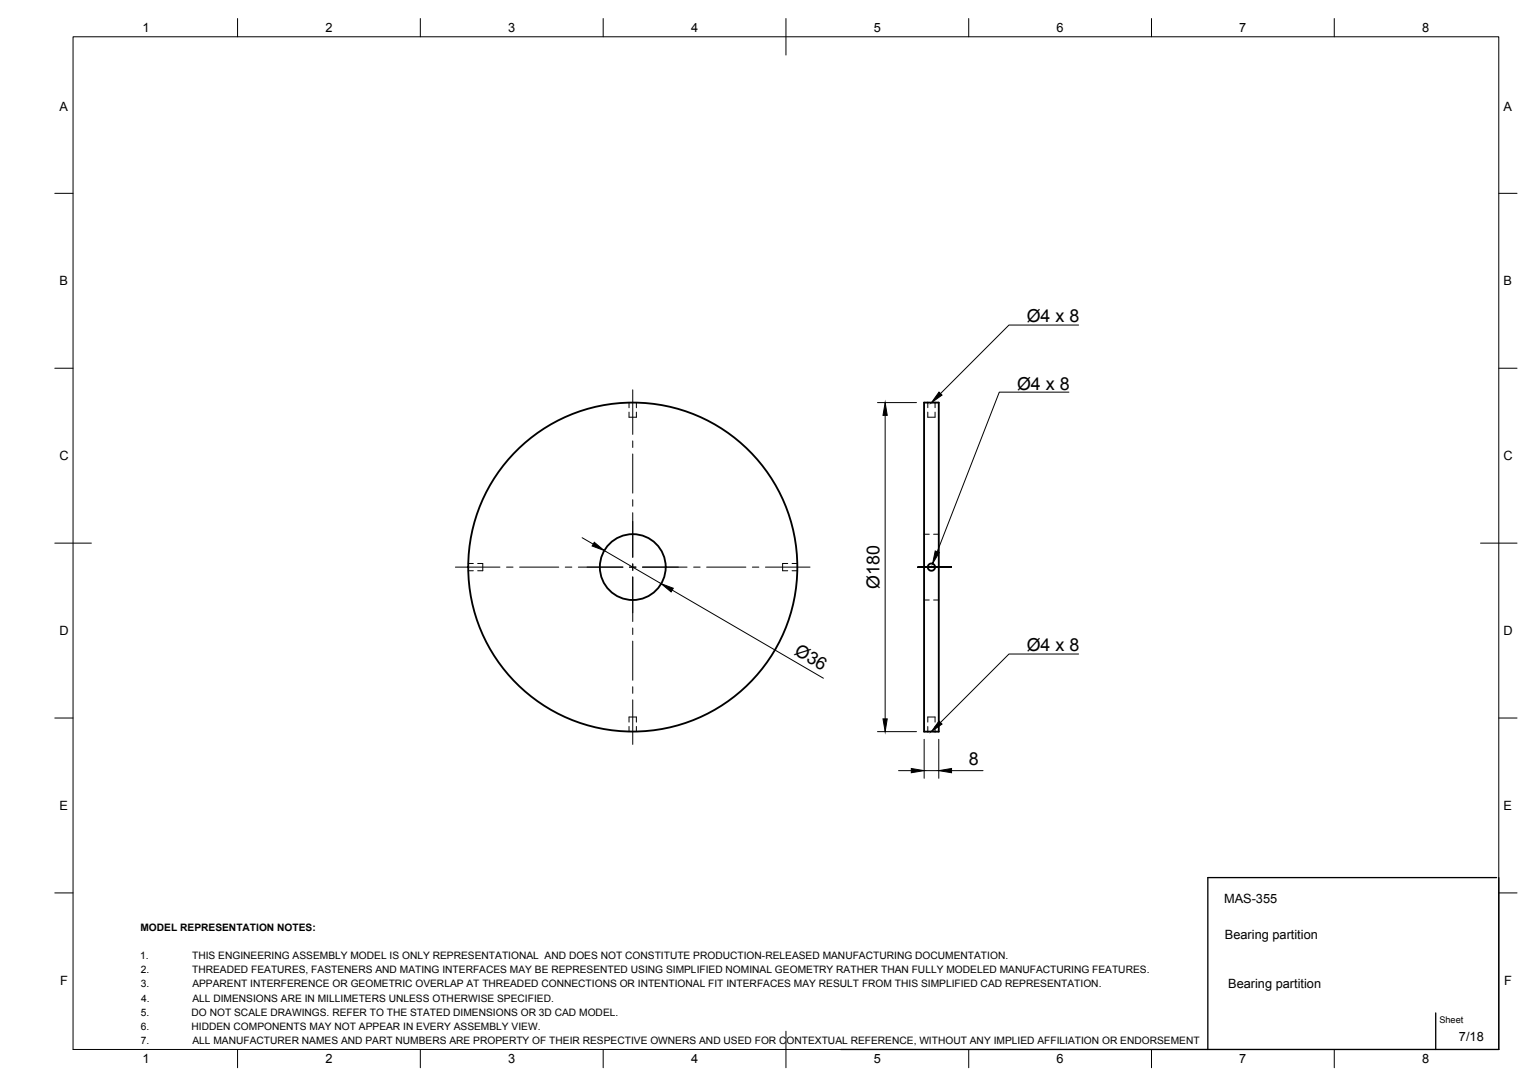
ISO-10303-21;
HEADER;
/* Generated by software containing ST-Developer
 * from STEP Tools, Inc. (www.steptools.com) 
 */

FILE_DESCRIPTION(
/* description */ ('Independent two-stage fixed-ring planetary gearbox,24/24/72 teeth,mod
ule2,20deg involutes,three planets per stage,4:1 x4:1=16:1. Native cut
-space/fillet/pattern tooth profiles derived from reusable gear blanks
; shared sun/planet/ring/carrier parts across both stages. Captured br
onze-journal input/carriers, headed retained planet pins, keyed inters
tage drive and modular keyed output interface. Native ideal gear links
; no torque, precision grade, production backlash/fits, lubrication, s
peed or life rating.'),
/* implementation_level */ '2;1');

FILE_NAME(
/* name */ 'Bearing partition.step',
/* time_stamp */ '2026-11-08T19:10:00-08:00',
/* author */ (''),
/* organization */ (''),
/* preprocessor_version */ 'ST-DEVELOPER v20.2',
/* originating_system */ 'Autodesk Translation Framework v15.17.0.0',
/* authorisation */ '');

FILE_SCHEMA (('AUTOMOTIVE_DESIGN { 1 0 10303 214 3 1 1 }'));
ENDSEC;

DATA;
#10=MECHANICAL_DESIGN_GEOMETRIC_PRESENTATION_REPRESENTATION('',(#1164),#259224);
#1124=SHAPE_REPRESENTATION_RELATIONSHIP('SRR','None',#259371,#1144);
#1144=ADVANCED_BREP_SHAPE_REPRESENTATION('',(#1184),#259205);
#1164=STYLED_ITEM('',(#259480),#1184);
#1184=MANIFOLD_SOLID_BREP('Body1',#25151);
#1242=FACE_BOUND('',#3407,.T.);
#1243=FACE_BOUND('',#3408,.T.);
#1244=FACE_BOUND('',#3409,.T.);
#1245=FACE_BOUND('',#3411,.T.);
#1246=FACE_BOUND('',#3413,.T.);
#1501=PLANE('',#25760);
#1502=PLANE('',#25763);
#1503=PLANE('',#25766);
#1504=PLANE('',#25769);
#1505=PLANE('',#25776);
#1506=PLANE('',#25777);
#2012=FACE_OUTER_BOUND('',#3397,.T.);
#2013=FACE_OUTER_BOUND('',#3398,.T.);
#2014=FACE_OUTER_BOUND('',#3399,.T.);
#2015=FACE_OUTER_BOUND('',#3400,.T.);
#2016=FACE_OUTER_BOUND('',#3401,.T.);
#2017=FACE_OUTER_BOUND('',#3402,.T.);
#2018=FACE_OUTER_BOUND('',#3403,.T.);
#2019=FACE_OUTER_BOUND('',#3404,.T.);
#2020=FACE_OUTER_BOUND('',#3405,.T.);
#2021=FACE_OUTER_BOUND('',#3406,.T.);
#2022=FACE_OUTER_BOUND('',#3410,.T.);
#2023=FACE_OUTER_BOUND('',#3412,.T.);
#3397=EDGE_LOOP('',(#17302,#17303,#17304,#17305,#17306));
#3398=EDGE_LOOP('',(#17307));
#3399=EDGE_LOOP('',(#17308,#17309,#17310,#17311,#17312));
#3400=EDGE_LOOP('',(#17313));
#3401=EDGE_LOOP('',(#17314,#17315,#17316,#17317,#17318,#17319));
#3402=EDGE_LOOP('',(#17320));
#3403=EDGE_LOOP('',(#17321,#17322,#17323,#17324,#17325,#17326));
#3404=EDGE_LOOP('',(#17327));
#3405=EDGE_LOOP('',(#17328,#17329,#17330,#17331));
#3406=EDGE_LOOP('',(#17332,#17333,#17334,#17335,#17336,#17337,#17338,#17339,
#17340));
#3407=EDGE_LOOP('',(#17341,#17342));
#3408=EDGE_LOOP('',(#17343,#17344));
#3409=EDGE_LOOP('',(#17345,#17346,#17347));
#3410=EDGE_LOOP('',(#17348));
#3411=EDGE_LOOP('',(#17349));
#3412=EDGE_LOOP('',(#17350));
#3413=EDGE_LOOP('',(#17351));
#4571=CIRCLE('',#25759,2.);
#4572=CIRCLE('',#25762,2.);
#4573=CIRCLE('',#25765,2.);
#4574=CIRCLE('',#25768,2.);
#4575=CIRCLE('',#25771,18.);
#4576=CIRCLE('',#25772,18.);
#4577=CIRCLE('',#25774,90.);
#4578=CIRCLE('',#25775,90.);
#5983=B_SPLINE_CURVE_WITH_KNOTS('',3,(#52036,#52037,#52038,#52039,#52040,
#52041,#52042,#52043,#52044,#52045,#52046,#52047,#52048,#52049,#52050,#52051,
#52052,#52053),.UNSPECIFIED.,.F.,.F.,(4,2,2,2,2,2,2,2,4),(0.301359994903926,
0.376699993319996,0.452039991736066,0.527379990771959,0.602719989807853,
0.678059988843746,0.753399987879639,0.828739986295709,0.904079984711779),
 .UNSPECIFIED.);
#5984=B_SPLINE_CURVE_WITH_KNOTS('',3,(#52057,#52058,#52059,#52060,#52061,
#52062,#52063,#52064,#52065,#52066,#52067,#52068,#52069,#52070,#52071,#52072,
#52073,#52074,#52075),.UNSPECIFIED.,.F.,.F.,(4,2,2,2,3,2,2,2,4),(0.904079984711779,
0.979419983127849,1.05475998154392,1.13009998057981,1.20543997961571,1.2807799786516,
1.35611997768749,1.43145997610356,1.50679997451963),.UNSPECIFIED.);
#5985=B_SPLINE_CURVE_WITH_KNOTS('',3,(#52080,#52081,#52082,#52083,#52084,
#52085,#52086,#52087,#52088,#52089,#52090,#52091,#52092,#52093,#52094,#52095,
#52096,#52097),.UNSPECIFIED.,.F.,.F.,(4,2,2,2,2,2,2,2,4),(0.301359994903926,
0.376699993319996,0.452039991736066,0.527379990771959,0.602719989807853,
0.678059988843746,0.753399987879639,0.828739986295709,0.904079984711779),
 .UNSPECIFIED.);
#5986=B_SPLINE_CURVE_WITH_KNOTS('',3,(#52098,#52099,#52100,#52101,#52102,
#52103,#52104,#52105,#52106,#52107,#52108,#52109,#52110,#52111,#52112,#52113,
#52114,#52115,#52116),.UNSPECIFIED.,.F.,.F.,(4,2,2,2,3,2,2,2,4),(0.904079984711779,
0.979419983127849,1.05475998154392,1.13009998057981,1.20543997961571,1.2807799786516,
1.35611997768749,1.43145997610356,1.50679997451963),.UNSPECIFIED.);
#5987=B_SPLINE_CURVE_WITH_KNOTS('',3,(#52124,#52125,#52126,#52127,#52128,
#52129,#52130,#52131,#52132,#52133,#52134,#52135,#52136,#52137,#52138,#52139,
#52140,#52141),.UNSPECIFIED.,.F.,.F.,(4,2,2,2,2,2,2,2,4),(0.301359994903926,
0.376699993319996,0.452039991736066,0.527379990771959,0.602719989807853,
0.678059988843746,0.753399987879639,0.828739986295709,0.904079984711779),
 .UNSPECIFIED.);
#5988=B_SPLINE_CURVE_WITH_KNOTS('',3,(#52143,#52144,#52145,#52146,#52147,
#52148,#52149,#52150,#52151,#52152),.UNSPECIFIED.,.F.,.F.,(4,2,2,2,4),(1.20543997961571,
1.2807799786516,1.35611997768749,1.43145997610356,1.50679997451963),
 .UNSPECIFIED.);
#5989=B_SPLINE_CURVE_WITH_KNOTS('',3,(#52156,#52157,#52158,#52159,#52160,
#52161,#52162,#52163,#52164,#52165),.UNSPECIFIED.,.F.,.F.,(4,2,2,2,4),(0.904079984711779,
0.979419983127849,1.05475998154392,1.13009998057981,1.20543997961571),
 .UNSPECIFIED.);
#5990=B_SPLINE_CURVE_WITH_KNOTS('',3,(#52170,#52171,#52172,#52173,#52174,
#52175,#52176,#52177,#52178,#52179,#52180,#52181,#52182,#52183,#52184,#52185,
#52186,#52187),.UNSPECIFIED.,.F.,.F.,(4,2,2,2,2,2,2,2,4),(0.301359994903926,
0.376699993319996,0.452039991736066,0.527379990771959,0.602719989807853,
0.678059988843746,0.753399987879639,0.828739986295709,0.904079984711779),
 .UNSPECIFIED.);
#5991=B_SPLINE_CURVE_WITH_KNOTS('',3,(#52189,#52190,#52191,#52192,#52193,
#52194,#52195,#52196,#52197,#52198),.UNSPECIFIED.,.F.,.F.,(4,2,2,2,4),(1.20543997961571,
1.2807799786516,1.35611997768749,1.43145997610356,1.50679997451963),
 .UNSPECIFIED.);
#5992=B_SPLINE_CURVE_WITH_KNOTS('',3,(#52202,#52203,#52204,#52205,#52206,
#52207,#52208,#52209,#52210,#52211),.UNSPECIFIED.,.F.,.F.,(4,2,2,2,4),(0.904079984711779,
0.979419983127849,1.05475998154392,1.13009998057981,1.20543997961571),
 .UNSPECIFIED.);
#6942=LINE('',#52055,#8127);
#6943=LINE('',#52118,#8128);
#6944=LINE('',#52154,#8129);
#6945=LINE('',#52200,#8130);
#6946=LINE('',#52217,#8131);
#6947=LINE('',#52222,#8132);
#6948=LINE('',#52224,#8133);
#8127=VECTOR('',#28345,2.);
#8128=VECTOR('',#28352,2.);
#8129=VECTOR('',#28359,2.);
#8130=VECTOR('',#28366,2.);
#8131=VECTOR('',#28375,18.);
#8132=VECTOR('',#28382,90.);
#8133=VECTOR('',#28383,90.);
#9669=VERTEX_POINT('',#52034);
#9670=VERTEX_POINT('',#52035);
#9671=VERTEX_POINT('',#52054);
#9672=VERTEX_POINT('',#52078);
#9673=VERTEX_POINT('',#52079);
#9674=VERTEX_POINT('',#52117);
#9675=VERTEX_POINT('',#52122);
#9676=VERTEX_POINT('',#52123);
#9677=VERTEX_POINT('',#52142);
#9678=VERTEX_POINT('',#52153);
#9679=VERTEX_POINT('',#52168);
#9680=VERTEX_POINT('',#52169);
#9681=VERTEX_POINT('',#52188);
#9682=VERTEX_POINT('',#52199);
#9683=VERTEX_POINT('',#52214);
#9684=VERTEX_POINT('',#52216);
#9685=VERTEX_POINT('',#52220);
#9686=VERTEX_POINT('',#52223);
#12536=EDGE_CURVE('',#9669,#9670,#5983,.T.);
#12537=EDGE_CURVE('',#9669,#9671,#6942,.T.);
#12538=EDGE_CURVE('',#9671,#9671,#4571,.T.);
#12539=EDGE_CURVE('',#9670,#9669,#5984,.T.);
#12540=EDGE_CURVE('',#9672,#9673,#5985,.T.);
#12541=EDGE_CURVE('',#9673,#9672,#5986,.T.);
#12542=EDGE_CURVE('',#9673,#9674,#6943,.T.);
#12543=EDGE_CURVE('',#9674,#9674,#4572,.T.);
#12544=EDGE_CURVE('',#9675,#9676,#5987,.T.);
#12545=EDGE_CURVE('',#9677,#9675,#5988,.T.);
#12546=EDGE_CURVE('',#9677,#9678,#6944,.T.);
#12547=EDGE_CURVE('',#9678,#9678,#4573,.T.);
#12548=EDGE_CURVE('',#9676,#9677,#5989,.T.);
#12549=EDGE_CURVE('',#9679,#9680,#5990,.T.);
#12550=EDGE_CURVE('',#9681,#9679,#5991,.T.);
#12551=EDGE_CURVE('',#9681,#9682,#6945,.T.);
#12552=EDGE_CURVE('',#9682,#9682,#4574,.T.);
#12553=EDGE_CURVE('',#9680,#9681,#5992,.T.);
#12554=EDGE_CURVE('',#9683,#9683,#4575,.T.);
#12555=EDGE_CURVE('',#9683,#9684,#6946,.T.);
#12556=EDGE_CURVE('',#9684,#9684,#4576,.T.);
#12557=EDGE_CURVE('',#9685,#9685,#4577,.T.);
#12558=EDGE_CURVE('',#9685,#9675,#6947,.T.);
#12559=EDGE_CURVE('',#9676,#9686,#6948,.T.);
#12560=EDGE_CURVE('',#9686,#9686,#4578,.T.);
#17302=ORIENTED_EDGE('',*,*,#12536,.F.);
#17303=ORIENTED_EDGE('',*,*,#12537,.T.);
#17304=ORIENTED_EDGE('',*,*,#12538,.T.);
#17305=ORIENTED_EDGE('',*,*,#12537,.F.);
#17306=ORIENTED_EDGE('',*,*,#12539,.F.);
#17307=ORIENTED_EDGE('',*,*,#12538,.F.);
#17308=ORIENTED_EDGE('',*,*,#12540,.F.);
#17309=ORIENTED_EDGE('',*,*,#12541,.F.);
#17310=ORIENTED_EDGE('',*,*,#12542,.T.);
#17311=ORIENTED_EDGE('',*,*,#12543,.T.);
#17312=ORIENTED_EDGE('',*,*,#12542,.F.);
#17313=ORIENTED_EDGE('',*,*,#12543,.F.);
#17314=ORIENTED_EDGE('',*,*,#12544,.F.);
#17315=ORIENTED_EDGE('',*,*,#12545,.F.);
#17316=ORIENTED_EDGE('',*,*,#12546,.T.);
#17317=ORIENTED_EDGE('',*,*,#12547,.T.);
#17318=ORIENTED_EDGE('',*,*,#12546,.F.);
#17319=ORIENTED_EDGE('',*,*,#12548,.F.);
#17320=ORIENTED_EDGE('',*,*,#12547,.F.);
#17321=ORIENTED_EDGE('',*,*,#12549,.F.);
#17322=ORIENTED_EDGE('',*,*,#12550,.F.);
#17323=ORIENTED_EDGE('',*,*,#12551,.T.);
#17324=ORIENTED_EDGE('',*,*,#12552,.T.);
#17325=ORIENTED_EDGE('',*,*,#12551,.F.);
#17326=ORIENTED_EDGE('',*,*,#12553,.F.);
#17327=ORIENTED_EDGE('',*,*,#12552,.F.);
#17328=ORIENTED_EDGE('',*,*,#12554,.F.);
#17329=ORIENTED_EDGE('',*,*,#12555,.T.);
#17330=ORIENTED_EDGE('',*,*,#12556,.T.);
#17331=ORIENTED_EDGE('',*,*,#12555,.F.);
#17332=ORIENTED_EDGE('',*,*,#12557,.F.);
#17333=ORIENTED_EDGE('',*,*,#12558,.T.);
#17334=ORIENTED_EDGE('',*,*,#12544,.T.);
#17335=ORIENTED_EDGE('',*,*,#12559,.T.);
#17336=ORIENTED_EDGE('',*,*,#12560,.T.);
#17337=ORIENTED_EDGE('',*,*,#12559,.F.);
#17338=ORIENTED_EDGE('',*,*,#12548,.T.);
#17339=ORIENTED_EDGE('',*,*,#12545,.T.);
#17340=ORIENTED_EDGE('',*,*,#12558,.F.);
#17341=ORIENTED_EDGE('',*,*,#12536,.T.);
#17342=ORIENTED_EDGE('',*,*,#12539,.T.);
#17343=ORIENTED_EDGE('',*,*,#12540,.T.);
#17344=ORIENTED_EDGE('',*,*,#12541,.T.);
#17345=ORIENTED_EDGE('',*,*,#12549,.T.);
#17346=ORIENTED_EDGE('',*,*,#12553,.T.);
#17347=ORIENTED_EDGE('',*,*,#12550,.T.);
#17348=ORIENTED_EDGE('',*,*,#12557,.T.);
#17349=ORIENTED_EDGE('',*,*,#12554,.T.);
#17350=ORIENTED_EDGE('',*,*,#12560,.F.);
#17351=ORIENTED_EDGE('',*,*,#12556,.F.);
#23355=CYLINDRICAL_SURFACE('',#25758,2.);
#23356=CYLINDRICAL_SURFACE('',#25761,2.);
#23357=CYLINDRICAL_SURFACE('',#25764,2.);
#23358=CYLINDRICAL_SURFACE('',#25767,2.);
#23359=CYLINDRICAL_SURFACE('',#25770,18.);
#23360=CYLINDRICAL_SURFACE('',#25773,90.);
#24118=ADVANCED_FACE('',(#2012),#23355,.F.);
#24119=ADVANCED_FACE('',(#2013),#1501,.F.);
#24120=ADVANCED_FACE('',(#2014),#23356,.F.);
#24121=ADVANCED_FACE('',(#2015),#1502,.F.);
#24122=ADVANCED_FACE('',(#2016),#23357,.F.);
#24123=ADVANCED_FACE('',(#2017),#1503,.F.);
#24124=ADVANCED_FACE('',(#2018),#23358,.F.);
#24125=ADVANCED_FACE('',(#2019),#1504,.F.);
#24126=ADVANCED_FACE('',(#2020),#23359,.F.);
#24127=ADVANCED_FACE('',(#2021,#1242,#1243,#1244),#23360,.T.);
#24128=ADVANCED_FACE('',(#2022,#1245),#1505,.T.);
#24129=ADVANCED_FACE('',(#2023,#1246),#1506,.F.);
#25151=CLOSED_SHELL('',(#24118,#24119,#24120,#24121,#24122,#24123,#24124,
#24125,#24126,#24127,#24128,#24129));
#25757=AXIS2_PLACEMENT_3D('',#52032,#28341,#28342);
#25758=AXIS2_PLACEMENT_3D('',#52033,#28343,#28344);
#25759=AXIS2_PLACEMENT_3D('',#52056,#28346,#28347);
#25760=AXIS2_PLACEMENT_3D('',#52076,#28348,#28349);
#25761=AXIS2_PLACEMENT_3D('',#52077,#28350,#28351);
#25762=AXIS2_PLACEMENT_3D('',#52119,#28353,#28354);
#25763=AXIS2_PLACEMENT_3D('',#52120,#28355,#28356);
#25764=AXIS2_PLACEMENT_3D('',#52121,#28357,#28358);
#25765=AXIS2_PLACEMENT_3D('',#52155,#28360,#28361);
#25766=AXIS2_PLACEMENT_3D('',#52166,#28362,#28363);
#25767=AXIS2_PLACEMENT_3D('',#52167,#28364,#28365);
#25768=AXIS2_PLACEMENT_3D('',#52201,#28367,#28368);
#25769=AXIS2_PLACEMENT_3D('',#52212,#28369,#28370);
#25770=AXIS2_PLACEMENT_3D('',#52213,#28371,#28372);
#25771=AXIS2_PLACEMENT_3D('',#52215,#28373,#28374);
#25772=AXIS2_PLACEMENT_3D('',#52218,#28376,#28377);
#25773=AXIS2_PLACEMENT_3D('',#52219,#28378,#28379);
#25774=AXIS2_PLACEMENT_3D('',#52221,#28380,#28381);
#25775=AXIS2_PLACEMENT_3D('',#52225,#28384,#28385);
#25776=AXIS2_PLACEMENT_3D('',#52226,#28386,#28387);
#25777=AXIS2_PLACEMENT_3D('',#52227,#28388,#28389);
#28341=DIRECTION('axis',(0.,0.,1.));
#28342=DIRECTION('refdir',(1.,0.,0.));
#28343=DIRECTION('center_axis',(0.,1.,0.));
#28344=DIRECTION('ref_axis',(0.,0.,-1.));
#28345=DIRECTION('',(0.,1.,0.));
#28346=DIRECTION('center_axis',(0.,1.,0.));
#28347=DIRECTION('ref_axis',(0.,0.,-1.));
#28348=DIRECTION('center_axis',(0.,1.,0.));
#28349=DIRECTION('ref_axis',(0.,0.,-1.));
#28350=DIRECTION('center_axis',(0.,-1.,0.));
#28351=DIRECTION('ref_axis',(0.,0.,1.));
#28352=DIRECTION('',(0.,-1.,0.));
#28353=DIRECTION('center_axis',(0.,-1.,0.));
#28354=DIRECTION('ref_axis',(0.,0.,1.));
#28355=DIRECTION('center_axis',(0.,-1.,0.));
#28356=DIRECTION('ref_axis',(0.,0.,1.));
#28357=DIRECTION('center_axis',(1.,0.,0.));
#28358=DIRECTION('ref_axis',(0.,-1.,0.));
#28359=DIRECTION('',(1.,0.,0.));
#28360=DIRECTION('center_axis',(1.,0.,0.));
#28361=DIRECTION('ref_axis',(0.,-1.,0.));
#28362=DIRECTION('center_axis',(1.,0.,0.));
#28363=DIRECTION('ref_axis',(0.,-1.,0.));
#28364=DIRECTION('center_axis',(-1.,0.,0.));
#28365=DIRECTION('ref_axis',(0.,1.,0.));
#28366=DIRECTION('',(-1.,0.,0.));
#28367=DIRECTION('center_axis',(-1.,0.,0.));
#28368=DIRECTION('ref_axis',(0.,1.,0.));
#28369=DIRECTION('center_axis',(-1.,0.,0.));
#28370=DIRECTION('ref_axis',(0.,1.,0.));
#28371=DIRECTION('center_axis',(0.,0.,1.));
#28372=DIRECTION('ref_axis',(1.,0.,0.));
#28373=DIRECTION('center_axis',(0.,0.,-1.));
#28374=DIRECTION('ref_axis',(1.,0.,0.));
#28375=DIRECTION('',(0.,0.,-1.));
#28376=DIRECTION('center_axis',(0.,0.,-1.));
#28377=DIRECTION('ref_axis',(1.,0.,0.));
#28378=DIRECTION('center_axis',(0.,0.,1.));
#28379=DIRECTION('ref_axis',(1.,0.,0.));
#28380=DIRECTION('center_axis',(0.,0.,1.));
#28381=DIRECTION('ref_axis',(1.,0.,0.));
#28382=DIRECTION('',(0.,0.,-1.));
#28383=DIRECTION('',(0.,0.,-1.));
#28384=DIRECTION('center_axis',(0.,0.,1.));
#28385=DIRECTION('ref_axis',(1.,0.,0.));
#28386=DIRECTION('center_axis',(0.,0.,1.));
#28387=DIRECTION('ref_axis',(1.,0.,0.));
#28388=DIRECTION('center_axis',(0.,0.,1.));
#28389=DIRECTION('ref_axis',(1.,0.,0.));
#52032=CARTESIAN_POINT('',(0.,0.,0.));
#52033=CARTESIAN_POINT('Origin',(0.,-86.,4.));
#52034=CARTESIAN_POINT('',(0.,-90.,6.));
#52035=CARTESIAN_POINT('',(0.,-90.,2.));
#52036=CARTESIAN_POINT('Ctrl Pts',(-2.08166817117217E-16,-90.,6.));
#52037=CARTESIAN_POINT('Ctrl Pts',(0.251133328053566,-90.,6.));
#52038=CARTESIAN_POINT('Ctrl Pts',(0.519000232590761,-89.9988407998655,
5.94980925763969));
#52039=CARTESIAN_POINT('Ctrl Pts',(1.01175644254643,-89.9946501491172,5.74569936791146));
#52040=CARTESIAN_POINT('Ctrl Pts',(1.23664644642618,-89.9916787455059,5.59178067832001));
#52041=CARTESIAN_POINT('Ctrl Pts',(1.59178067978086,-89.9860976603374,5.23664644496533));
#52042=CARTESIAN_POINT('Ctrl Pts',(1.74569936855887,-89.9831259365723,5.01175644187864));
#52043=CARTESIAN_POINT('Ctrl Pts',(1.94980925677131,-89.9789345539658,4.51900023379203));
#52044=CARTESIAN_POINT('Ctrl Pts',(2.,-89.9777750336159,4.25113333011964));
#52045=CARTESIAN_POINT('Ctrl Pts',(2.,-89.9777750336159,3.74886666988036));
#52046=CARTESIAN_POINT('Ctrl Pts',(1.94980925677131,-89.9789345539658,3.48099976620797));
#52047=CARTESIAN_POINT('Ctrl Pts',(1.74569936855887,-89.9831259365723,2.98824355812136));
#52048=CARTESIAN_POINT('Ctrl Pts',(1.59178067978086,-89.9860976603374,2.76335355503467));
#52049=CARTESIAN_POINT('Ctrl Pts',(1.23664644642618,-89.9916787455059,2.40821932167999));
#52050=CARTESIAN_POINT('Ctrl Pts',(1.01175644254643,-89.9946501491172,2.25430063208854));
#52051=CARTESIAN_POINT('Ctrl Pts',(0.519000232590762,-89.9988407998655,
2.05019074236031));
#52052=CARTESIAN_POINT('Ctrl Pts',(0.251133328053567,-90.,2.));
#52053=CARTESIAN_POINT('Ctrl Pts',(4.16333634234434E-16,-90.,2.));
#52054=CARTESIAN_POINT('',(2.44929359829471E-16,-82.,6.));
#52055=CARTESIAN_POINT('',(2.44929359829471E-16,-86.,6.));
#52056=CARTESIAN_POINT('Origin',(0.,-82.,4.));
#52057=CARTESIAN_POINT('Ctrl Pts',(4.16333634234434E-16,-90.,2.));
#52058=CARTESIAN_POINT('Ctrl Pts',(-0.251133328053566,-90.,2.));
#52059=CARTESIAN_POINT('Ctrl Pts',(-0.519000232590761,-89.9988407998655,
2.05019074236031));
#52060=CARTESIAN_POINT('Ctrl Pts',(-1.01175644254643,-89.9946501491172,
2.25430063208854));
#52061=CARTESIAN_POINT('Ctrl Pts',(-1.23664644642618,-89.9916787455059,
2.40821932167999));
#52062=CARTESIAN_POINT('Ctrl Pts',(-1.59178067978086,-89.9860976603374,
2.76335355503467));
#52063=CARTESIAN_POINT('Ctrl Pts',(-1.74569936855887,-89.9831259365723,
2.98824355812136));
#52064=CARTESIAN_POINT('Ctrl Pts',(-1.94980925677131,-89.9789345539658,
3.48099976620797));
#52065=CARTESIAN_POINT('Ctrl Pts',(-2.,-89.9777750336159,3.74886666988036));
#52066=CARTESIAN_POINT('Ctrl Pts',(-2.,-89.9777750336159,4.));
#52067=CARTESIAN_POINT('Ctrl Pts',(-2.,-89.9777750336159,4.25113333011964));
#52068=CARTESIAN_POINT('Ctrl Pts',(-1.94980925677131,-89.9789345539658,
4.51900023379203));
#52069=CARTESIAN_POINT('Ctrl Pts',(-1.74569936855887,-89.9831259365723,
5.01175644187864));
#52070=CARTESIAN_POINT('Ctrl Pts',(-1.59178067978086,-89.9860976603374,
5.23664644496533));
#52071=CARTESIAN_POINT('Ctrl Pts',(-1.23664644642618,-89.9916787455059,
5.59178067832001));
#52072=CARTESIAN_POINT('Ctrl Pts',(-1.01175644254643,-89.9946501491172,
5.74569936791146));
#52073=CARTESIAN_POINT('Ctrl Pts',(-0.519000232590762,-89.9988407998655,
5.94980925763969));
#52074=CARTESIAN_POINT('Ctrl Pts',(-0.251133328053566,-90.,6.));
#52075=CARTESIAN_POINT('Ctrl Pts',(-2.08166817117217E-16,-90.,6.));
#52076=CARTESIAN_POINT('Origin',(0.,-82.,4.));
#52077=CARTESIAN_POINT('Origin',(0.,86.,4.));
#52078=CARTESIAN_POINT('',(0.,90.,6.));
#52079=CARTESIAN_POINT('',(0.,90.,2.));
#52080=CARTESIAN_POINT('Ctrl Pts',(6.93889390390723E-17,90.,6.));
#52081=CARTESIAN_POINT('Ctrl Pts',(-0.251133328053566,90.,6.));
#52082=CARTESIAN_POINT('Ctrl Pts',(-0.519000232590761,89.9988407998655,
5.94980925763969));
#52083=CARTESIAN_POINT('Ctrl Pts',(-1.01175644254643,89.9946501491172,5.74569936791146));
#52084=CARTESIAN_POINT('Ctrl Pts',(-1.23664644642618,89.9916787455059,5.59178067832001));
#52085=CARTESIAN_POINT('Ctrl Pts',(-1.59178067978086,89.9860976603374,5.23664644496533));
#52086=CARTESIAN_POINT('Ctrl Pts',(-1.74569936855887,89.9831259365723,5.01175644187864));
#52087=CARTESIAN_POINT('Ctrl Pts',(-1.94980925677131,89.9789345539658,4.51900023379203));
#52088=CARTESIAN_POINT('Ctrl Pts',(-2.,89.9777750336159,4.25113333011964));
#52089=CARTESIAN_POINT('Ctrl Pts',(-2.,89.9777750336159,3.74886666988036));
#52090=CARTESIAN_POINT('Ctrl Pts',(-1.94980925677131,89.9789345539658,3.48099976620797));
#52091=CARTESIAN_POINT('Ctrl Pts',(-1.74569936855887,89.9831259365723,2.98824355812136));
#52092=CARTESIAN_POINT('Ctrl Pts',(-1.59178067978086,89.9860976603374,2.76335355503467));
#52093=CARTESIAN_POINT('Ctrl Pts',(-1.23664644642618,89.9916787455059,2.40821932167999));
#52094=CARTESIAN_POINT('Ctrl Pts',(-1.01175644254643,89.9946501491172,2.25430063208854));
#52095=CARTESIAN_POINT('Ctrl Pts',(-0.519000232590762,89.9988407998655,
2.05019074236031));
#52096=CARTESIAN_POINT('Ctrl Pts',(-0.251133328053567,90.,2.));
#52097=CARTESIAN_POINT('Ctrl Pts',(-4.16333634234434E-16,90.,2.));
#52098=CARTESIAN_POINT('Ctrl Pts',(-3.46944695195361E-16,90.,2.));
#52099=CARTESIAN_POINT('Ctrl Pts',(0.251133328053566,90.,2.));
#52100=CARTESIAN_POINT('Ctrl Pts',(0.519000232590762,89.9988407998655,2.05019074236031));
#52101=CARTESIAN_POINT('Ctrl Pts',(1.01175644254643,89.9946501491172,2.25430063208854));
#52102=CARTESIAN_POINT('Ctrl Pts',(1.23664644642618,89.9916787455059,2.40821932167999));
#52103=CARTESIAN_POINT('Ctrl Pts',(1.59178067978086,89.9860976603374,2.76335355503467));
#52104=CARTESIAN_POINT('Ctrl Pts',(1.74569936855886,89.9831259365723,2.98824355812136));
#52105=CARTESIAN_POINT('Ctrl Pts',(1.94980925677131,89.9789345539658,3.48099976620797));
#52106=CARTESIAN_POINT('Ctrl Pts',(2.,89.9777750336159,3.74886666988036));
#52107=CARTESIAN_POINT('Ctrl Pts',(2.,89.9777750336159,4.));
#52108=CARTESIAN_POINT('Ctrl Pts',(2.,89.9777750336159,4.25113333011964));
#52109=CARTESIAN_POINT('Ctrl Pts',(1.94980925677131,89.9789345539658,4.51900023379203));
#52110=CARTESIAN_POINT('Ctrl Pts',(1.74569936855887,89.9831259365723,5.01175644187864));
#52111=CARTESIAN_POINT('Ctrl Pts',(1.59178067978086,89.9860976603374,5.23664644496533));
#52112=CARTESIAN_POINT('Ctrl Pts',(1.23664644642618,89.9916787455059,5.59178067832001));
#52113=CARTESIAN_POINT('Ctrl Pts',(1.01175644254643,89.9946501491172,5.74569936791146));
#52114=CARTESIAN_POINT('Ctrl Pts',(0.519000232590761,89.9988407998655,5.94980925763969));
#52115=CARTESIAN_POINT('Ctrl Pts',(0.251133328053566,90.,6.));
#52116=CARTESIAN_POINT('Ctrl Pts',(-6.93889390390723E-17,90.,6.));
#52117=CARTESIAN_POINT('',(2.44929359829471E-16,82.,2.));
#52118=CARTESIAN_POINT('',(2.44929359829471E-16,86.,2.));
#52119=CARTESIAN_POINT('Origin',(0.,82.,4.));
#52120=CARTESIAN_POINT('Origin',(0.,82.,4.));
#52121=CARTESIAN_POINT('Origin',(-86.,0.,4.));
#52122=CARTESIAN_POINT('',(-90.,0.,6.));
#52123=CARTESIAN_POINT('',(-90.,0.,2.));
#52124=CARTESIAN_POINT('Ctrl Pts',(-90.,4.16333634234434E-16,6.));
#52125=CARTESIAN_POINT('Ctrl Pts',(-90.,-0.251133328053566,6.));
#52126=CARTESIAN_POINT('Ctrl Pts',(-89.9988407998655,-0.519000232590761,
5.94980925763969));
#52127=CARTESIAN_POINT('Ctrl Pts',(-89.9946501491172,-1.01175644254643,
5.74569936791146));
#52128=CARTESIAN_POINT('Ctrl Pts',(-89.9916787455059,-1.23664644642618,
5.59178067832001));
#52129=CARTESIAN_POINT('Ctrl Pts',(-89.9860976603374,-1.59178067978086,
5.23664644496533));
#52130=CARTESIAN_POINT('Ctrl Pts',(-89.9831259365723,-1.74569936855887,
5.01175644187864));
#52131=CARTESIAN_POINT('Ctrl Pts',(-89.9789345539658,-1.94980925677131,
4.51900023379203));
#52132=CARTESIAN_POINT('Ctrl Pts',(-89.9777750336159,-2.,4.25113333011964));
#52133=CARTESIAN_POINT('Ctrl Pts',(-89.9777750336159,-2.,3.74886666988036));
#52134=CARTESIAN_POINT('Ctrl Pts',(-89.9789345539658,-1.94980925677131,
3.48099976620797));
#52135=CARTESIAN_POINT('Ctrl Pts',(-89.9831259365723,-1.74569936855887,
2.98824355812136));
#52136=CARTESIAN_POINT('Ctrl Pts',(-89.9860976603374,-1.59178067978086,
2.76335355503467));
#52137=CARTESIAN_POINT('Ctrl Pts',(-89.9916787455059,-1.23664644642618,
2.40821932167999));
#52138=CARTESIAN_POINT('Ctrl Pts',(-89.9946501491172,-1.01175644254643,
2.25430063208854));
#52139=CARTESIAN_POINT('Ctrl Pts',(-89.9988407998655,-0.519000232590762,
2.05019074236031));
#52140=CARTESIAN_POINT('Ctrl Pts',(-90.,-0.251133328053567,2.));
#52141=CARTESIAN_POINT('Ctrl Pts',(-90.,-5.55111512312578E-16,2.));
#52142=CARTESIAN_POINT('',(-89.9777750336159,2.,4.));
#52143=CARTESIAN_POINT('Ctrl Pts',(-89.9777750336159,2.,4.));
#52144=CARTESIAN_POINT('Ctrl Pts',(-89.9777750336159,2.,4.25113333011964));
#52145=CARTESIAN_POINT('Ctrl Pts',(-89.9789345539658,1.94980925677131,4.51900023379203));
#52146=CARTESIAN_POINT('Ctrl Pts',(-89.9831259365723,1.74569936855887,5.01175644187864));
#52147=CARTESIAN_POINT('Ctrl Pts',(-89.9860976603374,1.59178067978086,5.23664644496533));
#52148=CARTESIAN_POINT('Ctrl Pts',(-89.9916787455059,1.23664644642618,5.59178067832001));
#52149=CARTESIAN_POINT('Ctrl Pts',(-89.9946501491172,1.01175644254643,5.74569936791146));
#52150=CARTESIAN_POINT('Ctrl Pts',(-89.9988407998655,0.519000232590762,
5.94980925763969));
#52151=CARTESIAN_POINT('Ctrl Pts',(-90.,0.251133328053567,6.));
#52152=CARTESIAN_POINT('Ctrl Pts',(-90.,2.77555756156289E-16,6.));
#52153=CARTESIAN_POINT('',(-82.,2.,4.));
#52154=CARTESIAN_POINT('',(-86.,2.,4.));
#52155=CARTESIAN_POINT('Origin',(-82.,0.,4.));
#52156=CARTESIAN_POINT('Ctrl Pts',(-90.,-4.85722573273506E-16,2.));
#52157=CARTESIAN_POINT('Ctrl Pts',(-90.,0.251133328053565,2.));
#52158=CARTESIAN_POINT('Ctrl Pts',(-89.9988407998655,0.519000232590761,
2.05019074236031));
#52159=CARTESIAN_POINT('Ctrl Pts',(-89.9946501491172,1.01175644254643,2.25430063208854));
#52160=CARTESIAN_POINT('Ctrl Pts',(-89.9916787455059,1.23664644642618,2.40821932167999));
#52161=CARTESIAN_POINT('Ctrl Pts',(-89.9860976603374,1.59178067978086,2.76335355503467));
#52162=CARTESIAN_POINT('Ctrl Pts',(-89.9831259365723,1.74569936855886,2.98824355812136));
#52163=CARTESIAN_POINT('Ctrl Pts',(-89.9789345539658,1.94980925677131,3.48099976620797));
#52164=CARTESIAN_POINT('Ctrl Pts',(-89.9777750336159,2.,3.74886666988036));
#52165=CARTESIAN_POINT('Ctrl Pts',(-89.9777750336159,2.,4.));
#52166=CARTESIAN_POINT('Origin',(-82.,0.,4.));
#52167=CARTESIAN_POINT('Origin',(86.,0.,4.));
#52168=CARTESIAN_POINT('',(90.,0.,6.));
#52169=CARTESIAN_POINT('',(90.,0.,2.));
#52170=CARTESIAN_POINT('Ctrl Pts',(90.,-4.16333634234434E-16,6.));
#52171=CARTESIAN_POINT('Ctrl Pts',(90.,0.251133328053566,6.));
#52172=CARTESIAN_POINT('Ctrl Pts',(89.9988407998655,0.519000232590761,5.94980925763969));
#52173=CARTESIAN_POINT('Ctrl Pts',(89.9946501491172,1.01175644254643,5.74569936791146));
#52174=CARTESIAN_POINT('Ctrl Pts',(89.9916787455059,1.23664644642618,5.59178067832001));
#52175=CARTESIAN_POINT('Ctrl Pts',(89.9860976603374,1.59178067978086,5.23664644496533));
#52176=CARTESIAN_POINT('Ctrl Pts',(89.9831259365723,1.74569936855887,5.01175644187864));
#52177=CARTESIAN_POINT('Ctrl Pts',(89.9789345539658,1.94980925677131,4.51900023379203));
#52178=CARTESIAN_POINT('Ctrl Pts',(89.9777750336159,2.,4.25113333011964));
#52179=CARTESIAN_POINT('Ctrl Pts',(89.9777750336159,2.,3.74886666988036));
#52180=CARTESIAN_POINT('Ctrl Pts',(89.9789345539658,1.94980925677131,3.48099976620797));
#52181=CARTESIAN_POINT('Ctrl Pts',(89.9831259365723,1.74569936855887,2.98824355812136));
#52182=CARTESIAN_POINT('Ctrl Pts',(89.9860976603374,1.59178067978086,2.76335355503467));
#52183=CARTESIAN_POINT('Ctrl Pts',(89.9916787455059,1.23664644642618,2.40821932167999));
#52184=CARTESIAN_POINT('Ctrl Pts',(89.9946501491172,1.01175644254643,2.25430063208854));
#52185=CARTESIAN_POINT('Ctrl Pts',(89.9988407998655,0.519000232590762,2.05019074236031));
#52186=CARTESIAN_POINT('Ctrl Pts',(90.,0.251133328053567,2.));
#52187=CARTESIAN_POINT('Ctrl Pts',(90.,5.55111512312578E-16,2.));
#52188=CARTESIAN_POINT('',(89.9777750336159,-2.,4.));
#52189=CARTESIAN_POINT('Ctrl Pts',(89.9777750336159,-2.,4.));
#52190=CARTESIAN_POINT('Ctrl Pts',(89.9777750336159,-2.,4.25113333011964));
#52191=CARTESIAN_POINT('Ctrl Pts',(89.9789345539658,-1.94980925677131,4.51900023379203));
#52192=CARTESIAN_POINT('Ctrl Pts',(89.9831259365723,-1.74569936855887,5.01175644187864));
#52193=CARTESIAN_POINT('Ctrl Pts',(89.9860976603374,-1.59178067978086,5.23664644496533));
#52194=CARTESIAN_POINT('Ctrl Pts',(89.9916787455059,-1.23664644642618,5.59178067832001));
#52195=CARTESIAN_POINT('Ctrl Pts',(89.9946501491172,-1.01175644254643,5.74569936791146));
#52196=CARTESIAN_POINT('Ctrl Pts',(89.9988407998655,-0.519000232590762,
5.94980925763969));
#52197=CARTESIAN_POINT('Ctrl Pts',(90.,-0.251133328053567,6.));
#52198=CARTESIAN_POINT('Ctrl Pts',(90.,-2.77555756156289E-16,6.));
#52199=CARTESIAN_POINT('',(82.,-2.,4.));
#52200=CARTESIAN_POINT('',(86.,-2.,4.));
#52201=CARTESIAN_POINT('Origin',(82.,0.,4.));
#52202=CARTESIAN_POINT('Ctrl Pts',(90.,4.85722573273506E-16,2.));
#52203=CARTESIAN_POINT('Ctrl Pts',(90.,-0.251133328053565,2.));
#52204=CARTESIAN_POINT('Ctrl Pts',(89.9988407998655,-0.519000232590761,
2.05019074236031));
#52205=CARTESIAN_POINT('Ctrl Pts',(89.9946501491172,-1.01175644254643,2.25430063208854));
#52206=CARTESIAN_POINT('Ctrl Pts',(89.9916787455059,-1.23664644642618,2.40821932167999));
#52207=CARTESIAN_POINT('Ctrl Pts',(89.9860976603374,-1.59178067978086,2.76335355503467));
#52208=CARTESIAN_POINT('Ctrl Pts',(89.9831259365723,-1.74569936855886,2.98824355812136));
#52209=CARTESIAN_POINT('Ctrl Pts',(89.9789345539658,-1.94980925677131,3.48099976620797));
#52210=CARTESIAN_POINT('Ctrl Pts',(89.9777750336159,-2.,3.74886666988036));
#52211=CARTESIAN_POINT('Ctrl Pts',(89.9777750336159,-2.,4.));
#52212=CARTESIAN_POINT('Origin',(82.,0.,4.));
#52213=CARTESIAN_POINT('Origin',(0.,0.,0.));
#52214=CARTESIAN_POINT('',(-18.,-2.20436423846524E-15,8.));
#52215=CARTESIAN_POINT('Origin',(0.,0.,8.));
#52216=CARTESIAN_POINT('',(-18.,-2.20436423846524E-15,0.));
#52217=CARTESIAN_POINT('',(-18.,-2.20436423846524E-15,0.));
#52218=CARTESIAN_POINT('Origin',(0.,0.,0.));
#52219=CARTESIAN_POINT('Origin',(0.,0.,0.));
#52220=CARTESIAN_POINT('',(-90.,-1.10218211923262E-14,8.));
#52221=CARTESIAN_POINT('Origin',(0.,0.,8.));
#52222=CARTESIAN_POINT('',(-90.,-1.10218211923262E-14,0.));
#52223=CARTESIAN_POINT('',(-90.,-1.10218211923262E-14,0.));
#52224=CARTESIAN_POINT('',(-90.,-1.10218211923262E-14,0.));
#52225=CARTESIAN_POINT('Origin',(0.,0.,0.));
#52226=CARTESIAN_POINT('Origin',(0.,0.,8.));
#52227=CARTESIAN_POINT('Origin',(0.,0.,0.));
#259183=UNCERTAINTY_MEASURE_WITH_UNIT(LENGTH_MEASURE(0.01),#259225,
'DISTANCE_ACCURACY_VALUE',
'Maximum model space distance between geometric entities at asserted c
onnectivities');
#259202=UNCERTAINTY_MEASURE_WITH_UNIT(LENGTH_MEASURE(0.01),#259225,
'DISTANCE_ACCURACY_VALUE',
'Maximum model space distance between geometric entities at asserted c
onnectivities');
#259205=(
GEOMETRIC_REPRESENTATION_CONTEXT(3)
GLOBAL_UNCERTAINTY_ASSIGNED_CONTEXT((#259183))
GLOBAL_UNIT_ASSIGNED_CONTEXT((#259225,#259227,#259228))
REPRESENTATION_CONTEXT('','3D')
);
#259224=(
GEOMETRIC_REPRESENTATION_CONTEXT(3)
GLOBAL_UNCERTAINTY_ASSIGNED_CONTEXT((#259202))
GLOBAL_UNIT_ASSIGNED_CONTEXT((#259225,#259227,#259228))
REPRESENTATION_CONTEXT('','3D')
);
#259225=(
LENGTH_UNIT()
NAMED_UNIT(*)
SI_UNIT(.MILLI.,.METRE.)
);
#259227=(
NAMED_UNIT(*)
PLANE_ANGLE_UNIT()
SI_UNIT($,.RADIAN.)
);
#259228=(
NAMED_UNIT(*)
SI_UNIT($,.STERADIAN.)
SOLID_ANGLE_UNIT()
);
#259231=SHAPE_DEFINITION_REPRESENTATION(#259252,#259371);
#259252=PRODUCT_DEFINITION_SHAPE('',$,#259393);
#259371=SHAPE_REPRESENTATION('',(#25757),#259205);
#259390=PRODUCT_DEFINITION_CONTEXT('part definition',#259455,'design');
#259393=PRODUCT_DEFINITION('Bearing partition','Bearing partition',#259414,
#259390);
#259414=PRODUCT_DEFINITION_FORMATION('',$,#259459);
#259455=APPLICATION_CONTEXT(
'Core Data for Automotive Mechanical Design Process');
#259456=PRODUCT_CONTEXT('part definition',#259455,'mechanical');
#259459=PRODUCT('Bearing partition','Bearing partition',$,(#259456));
#259480=PRESENTATION_STYLE_ASSIGNMENT((#259495));
#259495=SURFACE_STYLE_USAGE(.BOTH.,#259510);
#259510=SURFACE_SIDE_STYLE('',(#259525));
#259525=SURFACE_STYLE_FILL_AREA(#259540);
#259540=FILL_AREA_STYLE('Partition gray',(#259555));
#259555=FILL_AREA_STYLE_COLOUR('Partition gray',#259570);
#259570=COLOUR_RGB('Partition gray',0.407843137254902,0.447058823529412,
0.498039215686275);
ENDSEC;
END-ISO-10303-21;
